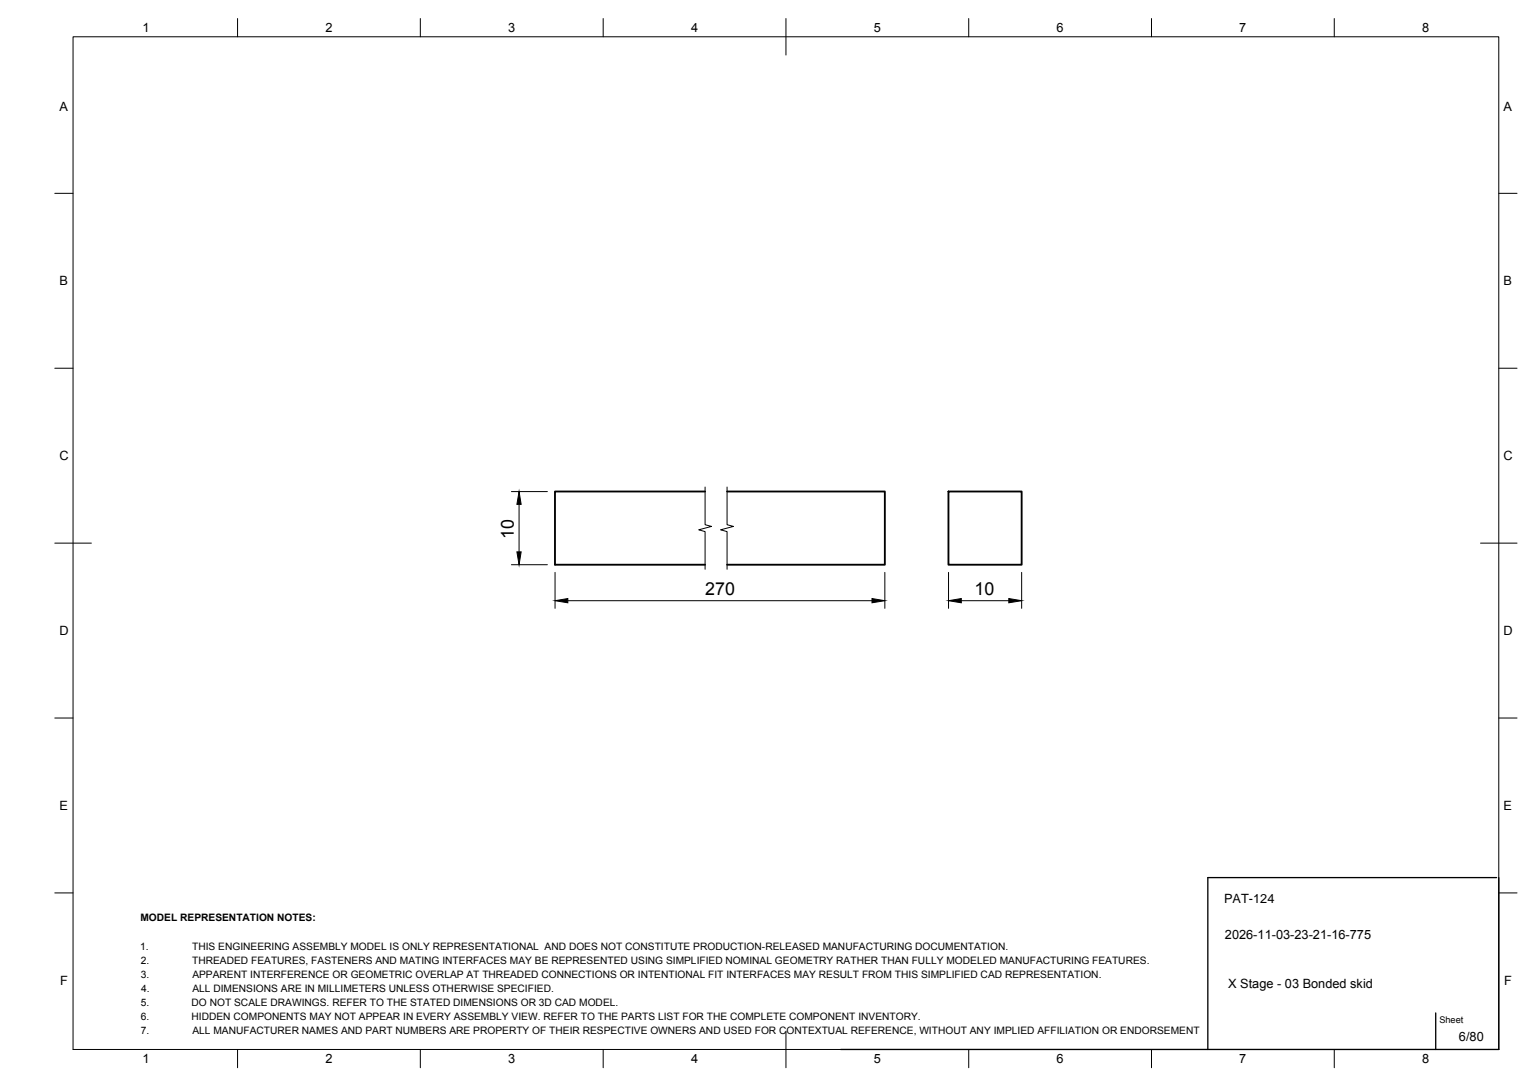
ISO-10303-21;
HEADER;
/* Generated by software containing ST-Developer
 * from STEP Tools, Inc. (www.steptools.com) 
 */

FILE_DESCRIPTION(
/* description */ ('XY cross-slide table'),
/* implementation_level */ '2;1');

FILE_NAME(
/* name */ 'X Stage - 03 Bonded skid.step',
/* time_stamp */ '2026-10-28T03:22:46-07:00',
/* author */ (''),
/* organization */ (''),
/* preprocessor_version */ 'ST-DEVELOPER v20.2',
/* originating_system */ 'Autodesk Translation Framework v15.17.0.0',
/* authorisation */ '');

FILE_SCHEMA (('AUTOMOTIVE_DESIGN { 1 0 10303 214 3 1 1 }'));
ENDSEC;

DATA;
#10=MECHANICAL_DESIGN_GEOMETRIC_PRESENTATION_REPRESENTATION('',(#1671),#62984);
#1505=SHAPE_REPRESENTATION_RELATIONSHIP('SRR','None',#63353,#1588);
#1588=ADVANCED_BREP_SHAPE_REPRESENTATION('',(#1784),#62890);
#1671=STYLED_ITEM('',(#63898),#1784);
#1784=MANIFOLD_SOLID_BREP('Body1',#22965);
#2302=PLANE('',#24041);
#2303=PLANE('',#24042);
#2304=PLANE('',#24043);
#2305=PLANE('',#24044);
#2306=PLANE('',#24045);
#2307=PLANE('',#24046);
#2885=FACE_OUTER_BOUND('',#4219,.T.);
#2886=FACE_OUTER_BOUND('',#4220,.T.);
#2887=FACE_OUTER_BOUND('',#4221,.T.);
#2888=FACE_OUTER_BOUND('',#4222,.T.);
#2889=FACE_OUTER_BOUND('',#4223,.T.);
#2890=FACE_OUTER_BOUND('',#4224,.T.);
#4219=EDGE_LOOP('',(#14988,#14989,#14990,#14991));
#4220=EDGE_LOOP('',(#14992,#14993,#14994,#14995));
#4221=EDGE_LOOP('',(#14996,#14997,#14998,#14999));
#4222=EDGE_LOOP('',(#15000,#15001,#15002,#15003));
#4223=EDGE_LOOP('',(#15004,#15005,#15006,#15007));
#4224=EDGE_LOOP('',(#15008,#15009,#15010,#15011));
#5928=LINE('',#32964,#7415);
#5929=LINE('',#32966,#7416);
#5930=LINE('',#32968,#7417);
#5931=LINE('',#32969,#7418);
#5932=LINE('',#32972,#7419);
#5933=LINE('',#32974,#7420);
#5934=LINE('',#32975,#7421);
#5935=LINE('',#32978,#7422);
#5936=LINE('',#32980,#7423);
#5937=LINE('',#32981,#7424);
#5938=LINE('',#32983,#7425);
#5939=LINE('',#32984,#7426);
#7415=VECTOR('',#26567,1.);
#7416=VECTOR('',#26568,1.);
#7417=VECTOR('',#26569,1.);
#7418=VECTOR('',#26570,1.);
#7419=VECTOR('',#26573,1.);
#7420=VECTOR('',#26574,1.);
#7421=VECTOR('',#26575,1.);
#7422=VECTOR('',#26578,1.);
#7423=VECTOR('',#26579,1.);
#7424=VECTOR('',#26580,1.);
#7425=VECTOR('',#26583,1.);
#7426=VECTOR('',#26584,1.);
#9801=VERTEX_POINT('',#32962);
#9802=VERTEX_POINT('',#32963);
#9803=VERTEX_POINT('',#32965);
#9804=VERTEX_POINT('',#32967);
#9805=VERTEX_POINT('',#32971);
#9806=VERTEX_POINT('',#32973);
#9807=VERTEX_POINT('',#32977);
#9808=VERTEX_POINT('',#32979);
#11878=EDGE_CURVE('',#9801,#9802,#5928,.T.);
#11879=EDGE_CURVE('',#9802,#9803,#5929,.T.);
#11880=EDGE_CURVE('',#9804,#9803,#5930,.T.);
#11881=EDGE_CURVE('',#9801,#9804,#5931,.T.);
#11882=EDGE_CURVE('',#9805,#9801,#5932,.T.);
#11883=EDGE_CURVE('',#9806,#9804,#5933,.T.);
#11884=EDGE_CURVE('',#9805,#9806,#5934,.T.);
#11885=EDGE_CURVE('',#9807,#9805,#5935,.T.);
#11886=EDGE_CURVE('',#9808,#9806,#5936,.T.);
#11887=EDGE_CURVE('',#9807,#9808,#5937,.T.);
#11888=EDGE_CURVE('',#9802,#9807,#5938,.T.);
#11889=EDGE_CURVE('',#9803,#9808,#5939,.T.);
#14988=ORIENTED_EDGE('',*,*,#11878,.T.);
#14989=ORIENTED_EDGE('',*,*,#11879,.T.);
#14990=ORIENTED_EDGE('',*,*,#11880,.F.);
#14991=ORIENTED_EDGE('',*,*,#11881,.F.);
#14992=ORIENTED_EDGE('',*,*,#11882,.T.);
#14993=ORIENTED_EDGE('',*,*,#11881,.T.);
#14994=ORIENTED_EDGE('',*,*,#11883,.F.);
#14995=ORIENTED_EDGE('',*,*,#11884,.F.);
#14996=ORIENTED_EDGE('',*,*,#11885,.T.);
#14997=ORIENTED_EDGE('',*,*,#11884,.T.);
#14998=ORIENTED_EDGE('',*,*,#11886,.F.);
#14999=ORIENTED_EDGE('',*,*,#11887,.F.);
#15000=ORIENTED_EDGE('',*,*,#11888,.T.);
#15001=ORIENTED_EDGE('',*,*,#11887,.T.);
#15002=ORIENTED_EDGE('',*,*,#11889,.F.);
#15003=ORIENTED_EDGE('',*,*,#11879,.F.);
#15004=ORIENTED_EDGE('',*,*,#11889,.T.);
#15005=ORIENTED_EDGE('',*,*,#11886,.T.);
#15006=ORIENTED_EDGE('',*,*,#11883,.T.);
#15007=ORIENTED_EDGE('',*,*,#11880,.T.);
#15008=ORIENTED_EDGE('',*,*,#11888,.F.);
#15009=ORIENTED_EDGE('',*,*,#11878,.F.);
#15010=ORIENTED_EDGE('',*,*,#11882,.F.);
#15011=ORIENTED_EDGE('',*,*,#11885,.F.);
#21666=ADVANCED_FACE('',(#2885),#2302,.T.);
#21667=ADVANCED_FACE('',(#2886),#2303,.T.);
#21668=ADVANCED_FACE('',(#2887),#2304,.T.);
#21669=ADVANCED_FACE('',(#2888),#2305,.T.);
#21670=ADVANCED_FACE('',(#2889),#2306,.T.);
#21671=ADVANCED_FACE('',(#2890),#2307,.F.);
#22965=CLOSED_SHELL('',(#21666,#21667,#21668,#21669,#21670,#21671));
#24040=AXIS2_PLACEMENT_3D('',#32960,#26563,#26564);
#24041=AXIS2_PLACEMENT_3D('',#32961,#26565,#26566);
#24042=AXIS2_PLACEMENT_3D('',#32970,#26571,#26572);
#24043=AXIS2_PLACEMENT_3D('',#32976,#26576,#26577);
#24044=AXIS2_PLACEMENT_3D('',#32982,#26581,#26582);
#24045=AXIS2_PLACEMENT_3D('',#32985,#26585,#26586);
#24046=AXIS2_PLACEMENT_3D('',#32986,#26587,#26588);
#26563=DIRECTION('axis',(0.,0.,1.));
#26564=DIRECTION('refdir',(1.,0.,0.));
#26565=DIRECTION('center_axis',(0.,1.,0.));
#26566=DIRECTION('ref_axis',(-1.,0.,0.));
#26567=DIRECTION('',(-1.,0.,0.));
#26568=DIRECTION('',(0.,0.,1.));
#26569=DIRECTION('',(-1.,0.,0.));
#26570=DIRECTION('',(0.,0.,1.));
#26571=DIRECTION('center_axis',(1.,0.,0.));
#26572=DIRECTION('ref_axis',(0.,1.,0.));
#26573=DIRECTION('',(0.,1.,0.));
#26574=DIRECTION('',(0.,1.,0.));
#26575=DIRECTION('',(0.,0.,1.));
#26576=DIRECTION('center_axis',(0.,-1.,0.));
#26577=DIRECTION('ref_axis',(1.,0.,0.));
#26578=DIRECTION('',(1.,0.,0.));
#26579=DIRECTION('',(1.,0.,0.));
#26580=DIRECTION('',(0.,0.,1.));
#26581=DIRECTION('center_axis',(-1.,0.,0.));
#26582=DIRECTION('ref_axis',(0.,-1.,0.));
#26583=DIRECTION('',(0.,-1.,0.));
#26584=DIRECTION('',(0.,-1.,0.));
#26585=DIRECTION('center_axis',(0.,0.,1.));
#26586=DIRECTION('ref_axis',(1.,0.,0.));
#26587=DIRECTION('center_axis',(0.,0.,1.));
#26588=DIRECTION('ref_axis',(1.,0.,0.));
#32960=CARTESIAN_POINT('',(0.,0.,0.));
#32961=CARTESIAN_POINT('Origin',(27.,-9.,-1.));
#32962=CARTESIAN_POINT('',(27.,-9.,-1.));
#32963=CARTESIAN_POINT('',(0.,-9.,-1.));
#32964=CARTESIAN_POINT('',(27.,-9.,-1.));
#32965=CARTESIAN_POINT('',(0.,-9.,0.));
#32966=CARTESIAN_POINT('',(0.,-9.,-1.));
#32967=CARTESIAN_POINT('',(27.,-9.,0.));
#32968=CARTESIAN_POINT('',(27.,-9.,0.));
#32969=CARTESIAN_POINT('',(27.,-9.,-1.));
#32970=CARTESIAN_POINT('Origin',(27.,-10.,-1.));
#32971=CARTESIAN_POINT('',(27.,-10.,-1.));
#32972=CARTESIAN_POINT('',(27.,-10.,-1.));
#32973=CARTESIAN_POINT('',(27.,-10.,0.));
#32974=CARTESIAN_POINT('',(27.,-10.,0.));
#32975=CARTESIAN_POINT('',(27.,-10.,-1.));
#32976=CARTESIAN_POINT('Origin',(0.,-10.,-1.));
#32977=CARTESIAN_POINT('',(0.,-10.,-1.));
#32978=CARTESIAN_POINT('',(0.,-10.,-1.));
#32979=CARTESIAN_POINT('',(0.,-10.,0.));
#32980=CARTESIAN_POINT('',(0.,-10.,0.));
#32981=CARTESIAN_POINT('',(0.,-10.,-1.));
#32982=CARTESIAN_POINT('Origin',(0.,-9.,-1.));
#32983=CARTESIAN_POINT('',(0.,-9.,-1.));
#32984=CARTESIAN_POINT('',(0.,-9.,0.));
#32985=CARTESIAN_POINT('Origin',(13.5,-9.5,0.));
#32986=CARTESIAN_POINT('Origin',(13.5,-9.5,-1.));
#62791=UNCERTAINTY_MEASURE_WITH_UNIT(LENGTH_MEASURE(0.001),#62985,
'DISTANCE_ACCURACY_VALUE',
'Maximum model space distance between geometric entities at asserted c
onnectivities');
#62885=UNCERTAINTY_MEASURE_WITH_UNIT(LENGTH_MEASURE(0.001),#62985,
'DISTANCE_ACCURACY_VALUE',
'Maximum model space distance between geometric entities at asserted c
onnectivities');
#62890=(
GEOMETRIC_REPRESENTATION_CONTEXT(3)
GLOBAL_UNCERTAINTY_ASSIGNED_CONTEXT((#62791))
GLOBAL_UNIT_ASSIGNED_CONTEXT((#62985,#62987,#62988))
REPRESENTATION_CONTEXT('','3D')
);
#62984=(
GEOMETRIC_REPRESENTATION_CONTEXT(3)
GLOBAL_UNCERTAINTY_ASSIGNED_CONTEXT((#62885))
GLOBAL_UNIT_ASSIGNED_CONTEXT((#62985,#62987,#62988))
REPRESENTATION_CONTEXT('','3D')
);
#62985=(
LENGTH_UNIT()
NAMED_UNIT(*)
SI_UNIT(.CENTI.,.METRE.)
);
#62987=(
NAMED_UNIT(*)
PLANE_ANGLE_UNIT()
SI_UNIT($,.RADIAN.)
);
#62988=(
NAMED_UNIT(*)
SI_UNIT($,.STERADIAN.)
SOLID_ANGLE_UNIT()
);
#62993=SHAPE_DEFINITION_REPRESENTATION(#63091,#63353);
#63091=PRODUCT_DEFINITION_SHAPE('',$,#63452);
#63353=SHAPE_REPRESENTATION('',(#24040),#62890);
#63447=PRODUCT_DEFINITION_CONTEXT('part definition',#63743,'design');
#63452=PRODUCT_DEFINITION('X Stage - 03 Bonded skid',
'X Stage - 03 Bonded skid',#63550,#63447);
#63550=PRODUCT_DEFINITION_FORMATION('',$,#63749);
#63743=APPLICATION_CONTEXT(
'Core Data for Automotive Mechanical Design Process');
#63744=PRODUCT_CONTEXT('part definition',#63743,'mechanical');
#63749=PRODUCT('X Stage - 03 Bonded skid','X Stage - 03 Bonded skid',
'X Stage - 03 Bonded skid',(#63744));
#63892=COLOUR_RGB('Light Blue',0.38,0.62,0.78);
#63893=FILL_AREA_STYLE_COLOUR('',#63892);
#63894=FILL_AREA_STYLE('',(#63893));
#63895=SURFACE_STYLE_FILL_AREA(#63894);
#63896=SURFACE_SIDE_STYLE('',(#63895));
#63897=SURFACE_STYLE_USAGE(.BOTH.,#63896);
#63898=PRESENTATION_STYLE_ASSIGNMENT((#63897));
ENDSEC;
END-ISO-10303-21;
